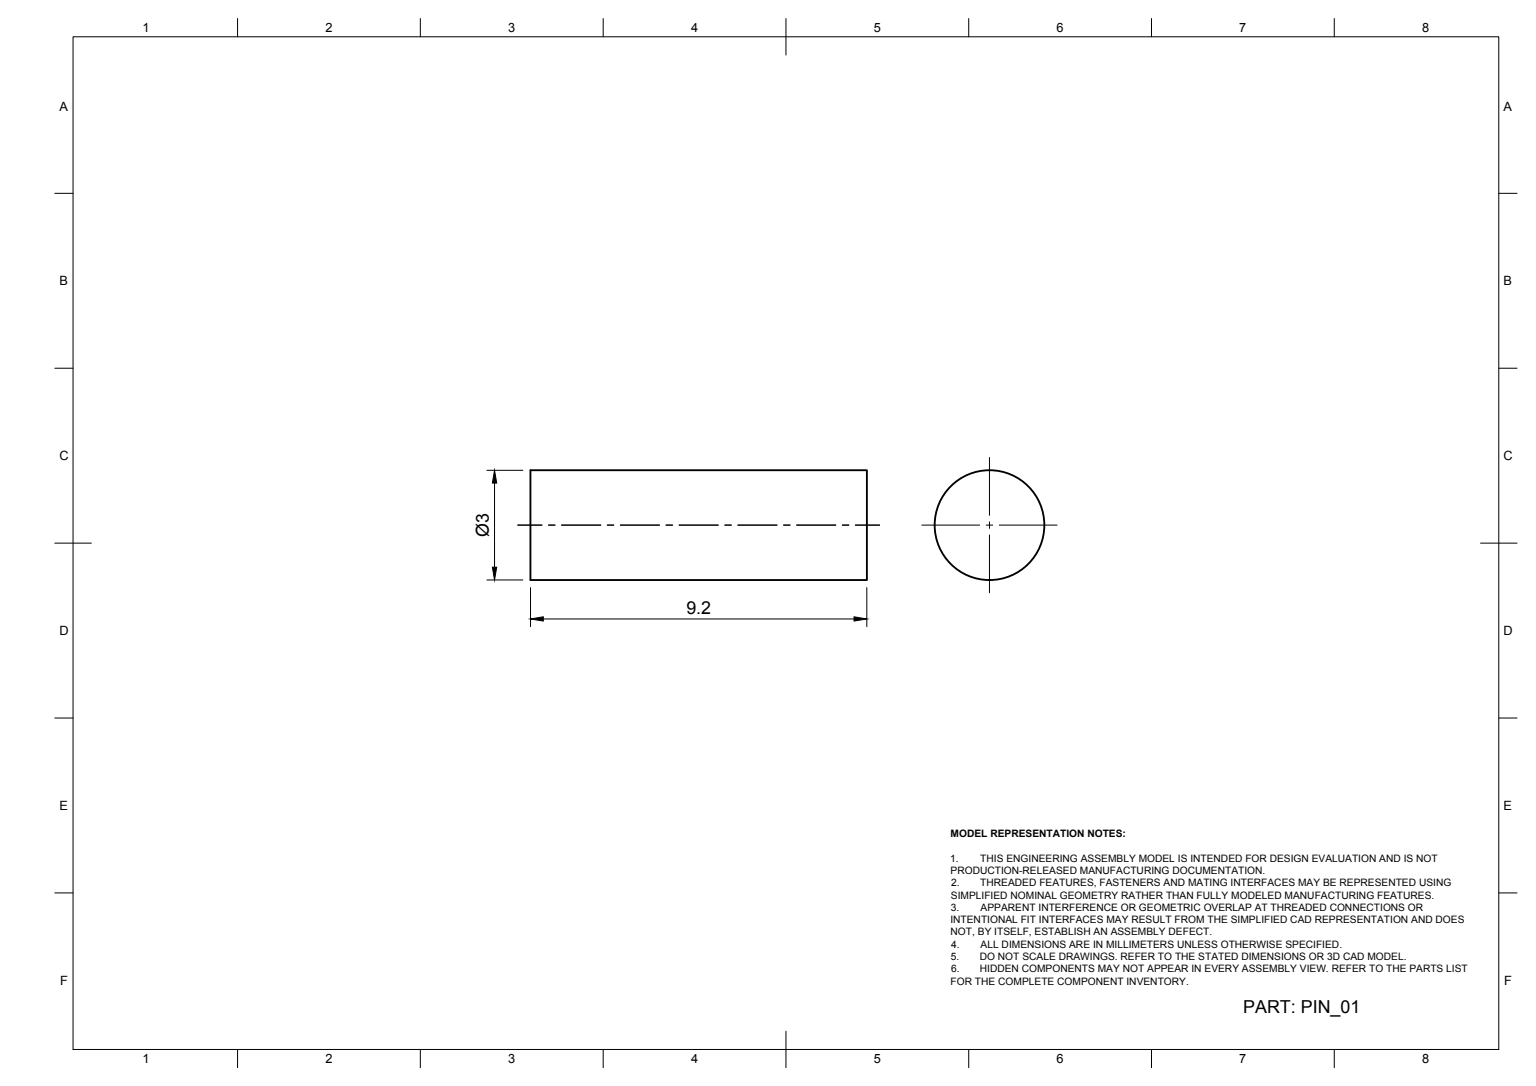
ISO-10303-21;
HEADER;
/* Generated by software containing ST-Developer
 * from STEP Tools, Inc. (www.steptools.com) 
 */

FILE_DESCRIPTION(
/* description */ (''),
/* implementation_level */ '2;1');

FILE_NAME(
/* name */ 'Pin_01.step',
/* time_stamp */ '2026-10-05T13:12:53-07:00',
/* author */ (''),
/* organization */ (''),
/* preprocessor_version */ 'ST-DEVELOPER v20.2',
/* originating_system */ 'Autodesk Translation Framework v15.15.0.0',
/* authorisation */ '');

FILE_SCHEMA (('AUTOMOTIVE_DESIGN { 1 0 10303 214 3 1 1 }'));
ENDSEC;

DATA;
#10=MECHANICAL_DESIGN_GEOMETRIC_PRESENTATION_REPRESENTATION('',(#61),#5912);
#45=SHAPE_REPRESENTATION_RELATIONSHIP('SRR','None',#5946,#53);
#53=ADVANCED_BREP_SHAPE_REPRESENTATION('',(#69),#5906);
#61=STYLED_ITEM('',(#5994),#69);
#69=MANIFOLD_SOLID_BREP('Body1',#3472);
#162=CYLINDRICAL_SURFACE('',#3845,1.50000013517123);
#332=FACE_OUTER_BOUND('',#535,.T.);
#333=FACE_OUTER_BOUND('',#536,.T.);
#334=FACE_OUTER_BOUND('',#537,.T.);
#535=EDGE_LOOP('',(#3124));
#536=EDGE_LOOP('',(#3125,#3126,#3127,#3128));
#537=EDGE_LOOP('',(#3129));
#643=CIRCLE('',#3844,1.50000013517123);
#644=CIRCLE('',#3846,1.50000013517123);
#1014=LINE('',#5838,#1379);
#1379=VECTOR('',#4805,1.50000013517123);
#1693=VERTEX_POINT('',#5833);
#1694=VERTEX_POINT('',#5836);
#2172=EDGE_CURVE('',#1693,#1693,#643,.T.);
#2173=EDGE_CURVE('',#1694,#1694,#644,.T.);
#2174=EDGE_CURVE('',#1694,#1693,#1014,.T.);
#3124=ORIENTED_EDGE('',*,*,#2172,.T.);
#3125=ORIENTED_EDGE('',*,*,#2173,.F.);
#3126=ORIENTED_EDGE('',*,*,#2174,.T.);
#3127=ORIENTED_EDGE('',*,*,#2172,.F.);
#3128=ORIENTED_EDGE('',*,*,#2174,.F.);
#3129=ORIENTED_EDGE('',*,*,#2173,.T.);
#3276=PLANE('',#3843);
#3277=PLANE('',#3847);
#3452=ADVANCED_FACE('',(#332),#3276,.F.);
#3453=ADVANCED_FACE('',(#333),#162,.T.);
#3454=ADVANCED_FACE('',(#334),#3277,.T.);
#3472=CLOSED_SHELL('',(#3452,#3453,#3454));
#3842=AXIS2_PLACEMENT_3D('',#5831,#4795,#4796);
#3843=AXIS2_PLACEMENT_3D('',#5832,#4797,#4798);
#3844=AXIS2_PLACEMENT_3D('',#5834,#4799,#4800);
#3845=AXIS2_PLACEMENT_3D('',#5835,#4801,#4802);
#3846=AXIS2_PLACEMENT_3D('',#5837,#4803,#4804);
#3847=AXIS2_PLACEMENT_3D('',#5839,#4806,#4807);
#4795=DIRECTION('axis',(0.,0.,1.));
#4796=DIRECTION('refdir',(1.,0.,0.));
#4797=DIRECTION('center_axis',(0.,-1.,0.));
#4798=DIRECTION('ref_axis',(1.,0.,0.));
#4799=DIRECTION('center_axis',(0.,1.,0.));
#4800=DIRECTION('ref_axis',(1.,0.,0.));
#4801=DIRECTION('center_axis',(0.,-1.,0.));
#4802=DIRECTION('ref_axis',(1.,0.,0.));
#4803=DIRECTION('center_axis',(0.,-1.,0.));
#4804=DIRECTION('ref_axis',(1.,0.,0.));
#4805=DIRECTION('',(0.,1.,0.));
#4806=DIRECTION('center_axis',(0.,-1.,0.));
#4807=DIRECTION('ref_axis',(1.,0.,0.));
#5831=CARTESIAN_POINT('',(0.,0.,0.));
#5832=CARTESIAN_POINT('Origin',(10.0000045479708,-2.8,103.499999046326));
#5833=CARTESIAN_POINT('',(8.50000441279955,-2.8,103.499999046326));
#5834=CARTESIAN_POINT('Origin',(10.0000045479708,-2.8,103.499999046326));
#5835=CARTESIAN_POINT('Origin',(10.0000045479708,-8.,103.499999046326));
#5836=CARTESIAN_POINT('',(8.50000441279955,-12.,103.499999046326));
#5837=CARTESIAN_POINT('Origin',(10.0000045479708,-12.,103.499999046326));
#5838=CARTESIAN_POINT('',(8.50000441279957,-8.,103.499999046326));
#5839=CARTESIAN_POINT('Origin',(10.0000045479708,-12.,103.499999046326));
#5896=UNCERTAINTY_MEASURE_WITH_UNIT(LENGTH_MEASURE(0.01),#5913,
'DISTANCE_ACCURACY_VALUE',
'Maximum model space distance between geometric entities at asserted c
onnectivities');
#5902=UNCERTAINTY_MEASURE_WITH_UNIT(LENGTH_MEASURE(0.01),#5913,
'DISTANCE_ACCURACY_VALUE',
'Maximum model space distance between geometric entities at asserted c
onnectivities');
#5906=(
GEOMETRIC_REPRESENTATION_CONTEXT(3)
GLOBAL_UNCERTAINTY_ASSIGNED_CONTEXT((#5896))
GLOBAL_UNIT_ASSIGNED_CONTEXT((#5913,#5915,#5916))
REPRESENTATION_CONTEXT('','3D')
);
#5912=(
GEOMETRIC_REPRESENTATION_CONTEXT(3)
GLOBAL_UNCERTAINTY_ASSIGNED_CONTEXT((#5902))
GLOBAL_UNIT_ASSIGNED_CONTEXT((#5913,#5915,#5916))
REPRESENTATION_CONTEXT('','3D')
);
#5913=(
LENGTH_UNIT()
NAMED_UNIT(*)
SI_UNIT(.MILLI.,.METRE.)
);
#5915=(
NAMED_UNIT(*)
PLANE_ANGLE_UNIT()
SI_UNIT($,.RADIAN.)
);
#5916=(
NAMED_UNIT(*)
SI_UNIT($,.STERADIAN.)
SOLID_ANGLE_UNIT()
);
#5920=SHAPE_DEFINITION_REPRESENTATION(#5929,#5946);
#5929=PRODUCT_DEFINITION_SHAPE('',$,#5956);
#5946=SHAPE_REPRESENTATION('',(#3842),#5906);
#5952=PRODUCT_DEFINITION_CONTEXT('part definition',#5981,'design');
#5956=PRODUCT_DEFINITION('Pin_01','Pin_01',#5965,#5952);
#5965=PRODUCT_DEFINITION_FORMATION('',$,#5986);
#5981=APPLICATION_CONTEXT(
'Core Data for Automotive Mechanical Design Process');
#5982=PRODUCT_CONTEXT('part definition',#5981,'mechanical');
#5986=PRODUCT('Pin_01','Pin_01',$,(#5982));
#5994=PRESENTATION_STYLE_ASSIGNMENT((#5997));
#5997=SURFACE_STYLE_USAGE(.BOTH.,#6000);
#6000=SURFACE_SIDE_STYLE('',(#6003));
#6003=SURFACE_STYLE_FILL_AREA(#6006);
#6006=FILL_AREA_STYLE('Opaque(160,160,160)',(#6009));
#6009=FILL_AREA_STYLE_COLOUR('Opaque(160,160,160)',#6012);
#6012=COLOUR_RGB('Opaque(160,160,160)', 0.31764706, 0.68627451, 0.89019608);
ENDSEC;
END-ISO-10303-21;
